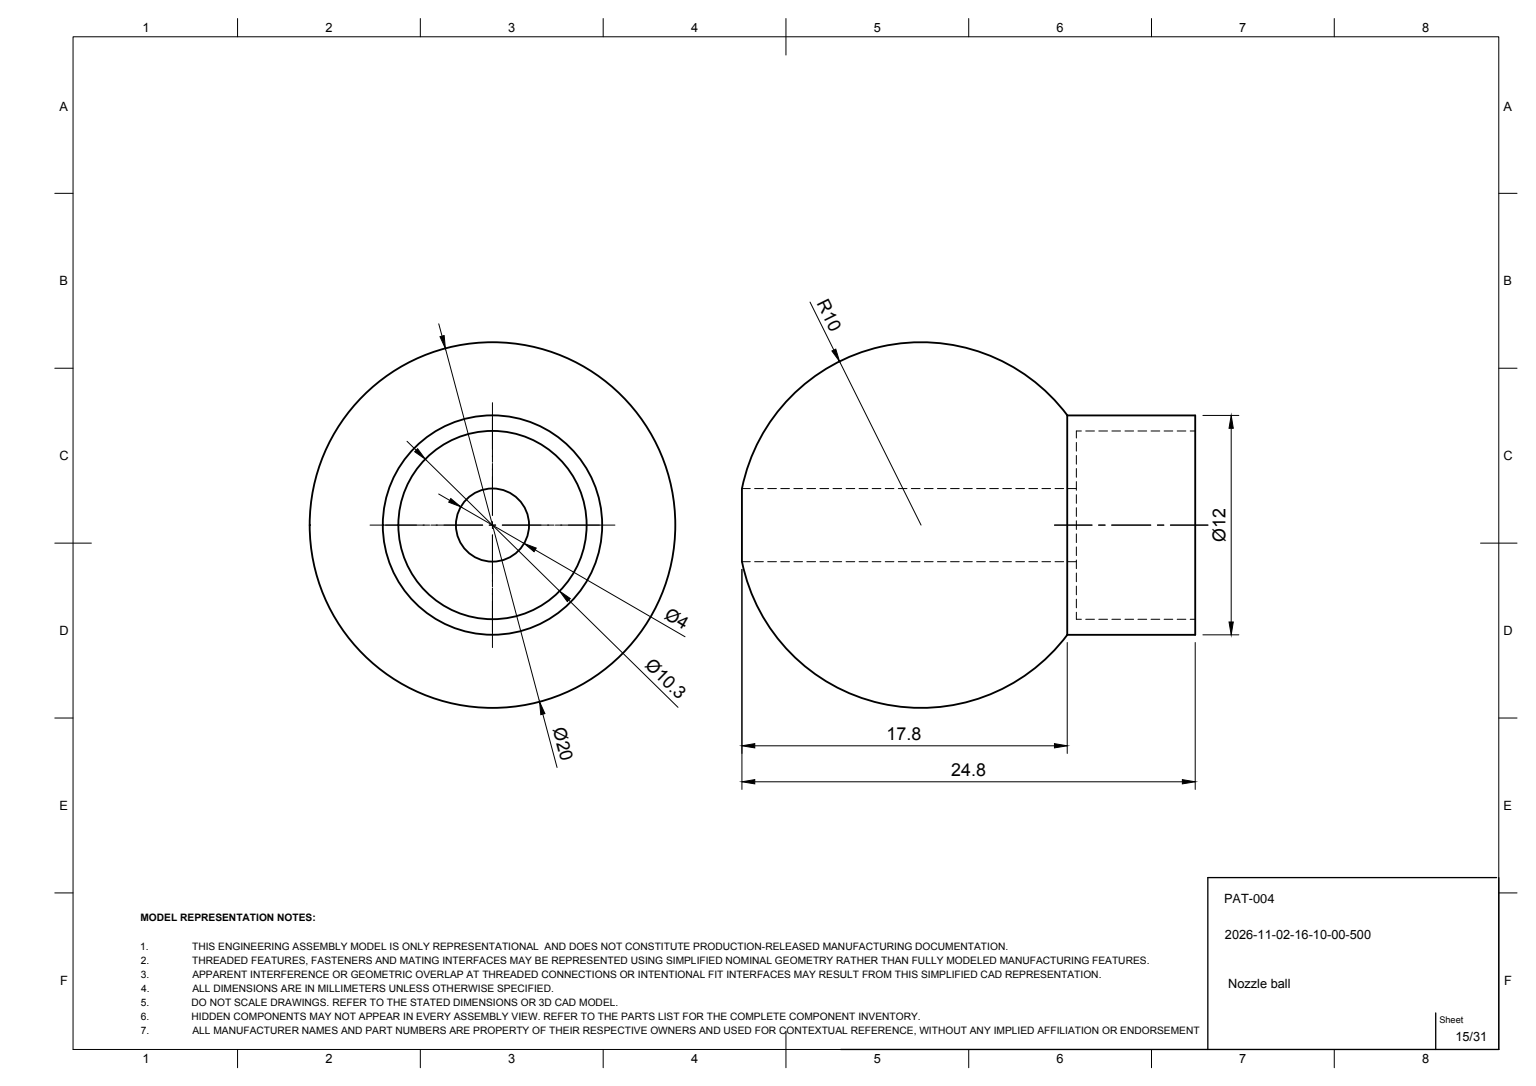
ISO-10303-21;
HEADER;
/* Generated by software containing ST-Developer
 * from STEP Tools, Inc. (www.steptools.com) 
 */

FILE_DESCRIPTION(
/* description */ ('Air blow-off nozzle station'),
/* implementation_level */ '2;1');

FILE_NAME(
/* name */ 'Nozzle ball.step',
/* time_stamp */ '2026-10-27T10:53:54-07:00',
/* author */ (''),
/* organization */ (''),
/* preprocessor_version */ 'ST-DEVELOPER v20.2',
/* originating_system */ 'Autodesk Translation Framework v15.17.0.0',
/* authorisation */ '');

FILE_SCHEMA (('AUTOMOTIVE_DESIGN { 1 0 10303 214 3 1 1 }'));
ENDSEC;

DATA;
#10=MECHANICAL_DESIGN_GEOMETRIC_PRESENTATION_REPRESENTATION('',(#251),#7897);
#168=SPHERICAL_SURFACE('',#4914,1.);
#201=SHAPE_REPRESENTATION_RELATIONSHIP('SRR','None',#8016,#226);
#226=ADVANCED_BREP_SHAPE_REPRESENTATION('',(#274),#7883);
#251=STYLED_ITEM('',(#8234),#274);
#274=MANIFOLD_SOLID_BREP('Body1',#4302);
#335=FACE_BOUND('',#1033,.T.);
#336=FACE_BOUND('',#1037,.T.);
#337=FACE_BOUND('',#1039,.T.);
#338=FACE_BOUND('',#1040,.T.);
#504=PLANE('',#4906);
#505=PLANE('',#4913);
#725=FACE_OUTER_BOUND('',#1031,.T.);
#726=FACE_OUTER_BOUND('',#1032,.T.);
#727=FACE_OUTER_BOUND('',#1034,.T.);
#728=FACE_OUTER_BOUND('',#1035,.T.);
#729=FACE_OUTER_BOUND('',#1036,.T.);
#730=FACE_OUTER_BOUND('',#1038,.T.);
#1031=EDGE_LOOP('',(#3725,#3726,#3727,#3728));
#1032=EDGE_LOOP('',(#3729));
#1033=EDGE_LOOP('',(#3730));
#1034=EDGE_LOOP('',(#3731,#3732,#3733,#3734));
#1035=EDGE_LOOP('',(#3735,#3736,#3737,#3738));
#1036=EDGE_LOOP('',(#3739));
#1037=EDGE_LOOP('',(#3740));
#1038=EDGE_LOOP('',(#3741,#3742));
#1039=EDGE_LOOP('',(#3743));
#1040=EDGE_LOOP('',(#3744));
#1442=LINE('',#7537,#1796);
#1443=LINE('',#7544,#1797);
#1444=LINE('',#7550,#1798);
#1796=VECTOR('',#6008,0.515);
#1797=VECTOR('',#6017,0.2);
#1798=VECTOR('',#6024,0.6);
#1940=CIRCLE('',#4904,0.515);
#1941=CIRCLE('',#4905,0.515);
#1942=CIRCLE('',#4907,0.2);
#1943=CIRCLE('',#4909,0.2);
#1944=CIRCLE('',#4911,0.6);
#1945=CIRCLE('',#4912,0.6);
#1946=CIRCLE('',#4915,1.);
#2284=VERTEX_POINT('',#7534);
#2285=VERTEX_POINT('',#7536);
#2286=VERTEX_POINT('',#7540);
#2287=VERTEX_POINT('',#7543);
#2288=VERTEX_POINT('',#7547);
#2289=VERTEX_POINT('',#7549);
#2290=VERTEX_POINT('',#7554);
#2291=VERTEX_POINT('',#7555);
#2780=EDGE_CURVE('',#2284,#2284,#1940,.T.);
#2781=EDGE_CURVE('',#2284,#2285,#1442,.T.);
#2782=EDGE_CURVE('',#2285,#2285,#1941,.T.);
#2783=EDGE_CURVE('',#2286,#2286,#1942,.T.);
#2784=EDGE_CURVE('',#2286,#2287,#1443,.T.);
#2785=EDGE_CURVE('',#2287,#2287,#1943,.T.);
#2786=EDGE_CURVE('',#2288,#2288,#1944,.T.);
#2787=EDGE_CURVE('',#2288,#2289,#1444,.T.);
#2788=EDGE_CURVE('',#2289,#2289,#1945,.T.);
#2789=EDGE_CURVE('',#2290,#2291,#1946,.T.);
#3725=ORIENTED_EDGE('',*,*,#2780,.F.);
#3726=ORIENTED_EDGE('',*,*,#2781,.T.);
#3727=ORIENTED_EDGE('',*,*,#2782,.T.);
#3728=ORIENTED_EDGE('',*,*,#2781,.F.);
#3729=ORIENTED_EDGE('',*,*,#2782,.F.);
#3730=ORIENTED_EDGE('',*,*,#2783,.F.);
#3731=ORIENTED_EDGE('',*,*,#2783,.T.);
#3732=ORIENTED_EDGE('',*,*,#2784,.T.);
#3733=ORIENTED_EDGE('',*,*,#2785,.F.);
#3734=ORIENTED_EDGE('',*,*,#2784,.F.);
#3735=ORIENTED_EDGE('',*,*,#2786,.F.);
#3736=ORIENTED_EDGE('',*,*,#2787,.T.);
#3737=ORIENTED_EDGE('',*,*,#2788,.T.);
#3738=ORIENTED_EDGE('',*,*,#2787,.F.);
#3739=ORIENTED_EDGE('',*,*,#2788,.F.);
#3740=ORIENTED_EDGE('',*,*,#2780,.T.);
#3741=ORIENTED_EDGE('',*,*,#2789,.T.);
#3742=ORIENTED_EDGE('',*,*,#2789,.F.);
#3743=ORIENTED_EDGE('',*,*,#2785,.T.);
#3744=ORIENTED_EDGE('',*,*,#2786,.T.);
#3998=CYLINDRICAL_SURFACE('',#4903,0.515);
#3999=CYLINDRICAL_SURFACE('',#4908,0.2);
#4000=CYLINDRICAL_SURFACE('',#4910,0.6);
#4215=ADVANCED_FACE('',(#725),#3998,.F.);
#4216=ADVANCED_FACE('',(#726,#335),#504,.F.);
#4217=ADVANCED_FACE('',(#727),#3999,.F.);
#4218=ADVANCED_FACE('',(#728),#4000,.T.);
#4219=ADVANCED_FACE('',(#729,#336),#505,.F.);
#4220=ADVANCED_FACE('',(#730,#337,#338),#168,.T.);
#4302=CLOSED_SHELL('',(#4215,#4216,#4217,#4218,#4219,#4220));
#4902=AXIS2_PLACEMENT_3D('',#7532,#6002,#6003);
#4903=AXIS2_PLACEMENT_3D('',#7533,#6004,#6005);
#4904=AXIS2_PLACEMENT_3D('',#7535,#6006,#6007);
#4905=AXIS2_PLACEMENT_3D('',#7538,#6009,#6010);
#4906=AXIS2_PLACEMENT_3D('',#7539,#6011,#6012);
#4907=AXIS2_PLACEMENT_3D('',#7541,#6013,#6014);
#4908=AXIS2_PLACEMENT_3D('',#7542,#6015,#6016);
#4909=AXIS2_PLACEMENT_3D('',#7545,#6018,#6019);
#4910=AXIS2_PLACEMENT_3D('',#7546,#6020,#6021);
#4911=AXIS2_PLACEMENT_3D('',#7548,#6022,#6023);
#4912=AXIS2_PLACEMENT_3D('',#7551,#6025,#6026);
#4913=AXIS2_PLACEMENT_3D('',#7552,#6027,#6028);
#4914=AXIS2_PLACEMENT_3D('',#7553,#6029,#6030);
#4915=AXIS2_PLACEMENT_3D('',#7556,#6031,#6032);
#6002=DIRECTION('axis',(0.,0.,1.));
#6003=DIRECTION('refdir',(1.,0.,0.));
#6004=DIRECTION('center_axis',(0.,1.,0.));
#6005=DIRECTION('ref_axis',(1.,0.,0.));
#6006=DIRECTION('center_axis',(0.,1.,0.));
#6007=DIRECTION('ref_axis',(1.,0.,0.));
#6008=DIRECTION('',(0.,1.,0.));
#6009=DIRECTION('center_axis',(0.,1.,0.));
#6010=DIRECTION('ref_axis',(1.,0.,0.));
#6011=DIRECTION('center_axis',(0.,1.,0.));
#6012=DIRECTION('ref_axis',(1.,0.,0.));
#6013=DIRECTION('center_axis',(0.,-1.,0.));
#6014=DIRECTION('ref_axis',(1.,0.,0.));
#6015=DIRECTION('center_axis',(0.,1.,0.));
#6016=DIRECTION('ref_axis',(1.,0.,0.));
#6017=DIRECTION('',(0.,1.,0.));
#6018=DIRECTION('center_axis',(0.,-1.,0.));
#6019=DIRECTION('ref_axis',(1.,-1.11022302462516E-15,0.));
#6020=DIRECTION('center_axis',(0.,1.,0.));
#6021=DIRECTION('ref_axis',(1.,0.,0.));
#6022=DIRECTION('center_axis',(0.,1.,0.));
#6023=DIRECTION('ref_axis',(1.,0.,0.));
#6024=DIRECTION('',(0.,-1.,0.));
#6025=DIRECTION('center_axis',(0.,1.,0.));
#6026=DIRECTION('ref_axis',(1.,0.,0.));
#6027=DIRECTION('center_axis',(0.,1.,0.));
#6028=DIRECTION('ref_axis',(1.,0.,0.));
#6029=DIRECTION('center_axis',(0.,0.,1.));
#6030=DIRECTION('ref_axis',(1.,0.,0.));
#6031=DIRECTION('center_axis',(0.,-1.,0.));
#6032=DIRECTION('ref_axis',(-1.,0.,0.));
#7532=CARTESIAN_POINT('',(0.,0.,0.));
#7533=CARTESIAN_POINT('Origin',(-3.,-3.6,23.));
#7534=CARTESIAN_POINT('',(-3.515,-3.5,23.));
#7535=CARTESIAN_POINT('Origin',(-3.,-3.5,23.));
#7536=CARTESIAN_POINT('',(-3.515,-2.85,23.));
#7537=CARTESIAN_POINT('',(-3.515,-3.6,23.));
#7538=CARTESIAN_POINT('Origin',(-3.,-2.85,23.));
#7539=CARTESIAN_POINT('Origin',(-3.,-2.85,23.));
#7540=CARTESIAN_POINT('',(-3.2,-2.85,23.));
#7541=CARTESIAN_POINT('Origin',(-3.,-2.85,23.));
#7542=CARTESIAN_POINT('Origin',(-3.,-3.6,23.));
#7543=CARTESIAN_POINT('',(-3.2,-1.02020410288673,23.));
#7544=CARTESIAN_POINT('',(-3.2,-3.6,23.));
#7545=CARTESIAN_POINT('Origin',(-3.,-1.02020410288673,23.));
#7546=CARTESIAN_POINT('Origin',(-3.,-3.5,23.));
#7547=CARTESIAN_POINT('',(-3.6,-2.8,23.));
#7548=CARTESIAN_POINT('Origin',(-3.,-2.8,23.));
#7549=CARTESIAN_POINT('',(-3.6,-3.5,23.));
#7550=CARTESIAN_POINT('',(-3.6,-3.5,23.));
#7551=CARTESIAN_POINT('Origin',(-3.,-3.5,23.));
#7552=CARTESIAN_POINT('Origin',(-3.,-3.5,23.));
#7553=CARTESIAN_POINT('Origin',(-3.,-2.,23.));
#7554=CARTESIAN_POINT('',(-3.,-2.,24.));
#7555=CARTESIAN_POINT('',(-3.,-2.,22.));
#7556=CARTESIAN_POINT('Origin',(-3.,-2.,23.));
#7851=UNCERTAINTY_MEASURE_WITH_UNIT(LENGTH_MEASURE(0.001),#7898,
'DISTANCE_ACCURACY_VALUE',
'Maximum model space distance between geometric entities at asserted c
onnectivities');
#7865=UNCERTAINTY_MEASURE_WITH_UNIT(LENGTH_MEASURE(0.001),#7898,
'DISTANCE_ACCURACY_VALUE',
'Maximum model space distance between geometric entities at asserted c
onnectivities');
#7883=(
GEOMETRIC_REPRESENTATION_CONTEXT(3)
GLOBAL_UNCERTAINTY_ASSIGNED_CONTEXT((#7851))
GLOBAL_UNIT_ASSIGNED_CONTEXT((#7898,#7900,#7901))
REPRESENTATION_CONTEXT('','3D')
);
#7897=(
GEOMETRIC_REPRESENTATION_CONTEXT(3)
GLOBAL_UNCERTAINTY_ASSIGNED_CONTEXT((#7865))
GLOBAL_UNIT_ASSIGNED_CONTEXT((#7898,#7900,#7901))
REPRESENTATION_CONTEXT('','3D')
);
#7898=(
LENGTH_UNIT()
NAMED_UNIT(*)
SI_UNIT(.CENTI.,.METRE.)
);
#7900=(
NAMED_UNIT(*)
PLANE_ANGLE_UNIT()
SI_UNIT($,.RADIAN.)
);
#7901=(
NAMED_UNIT(*)
SI_UNIT($,.STERADIAN.)
SOLID_ANGLE_UNIT()
);
#7919=SHAPE_DEFINITION_REPRESENTATION(#7967,#8016);
#7967=PRODUCT_DEFINITION_SHAPE('',$,#8048);
#8016=SHAPE_REPRESENTATION('',(#4902),#7883);
#8030=PRODUCT_DEFINITION_CONTEXT('part definition',#8125,'design');
#8048=PRODUCT_DEFINITION('Nozzle ball','Nozzle ball',#8079,#8030);
#8079=PRODUCT_DEFINITION_FORMATION('',$,#8144);
#8125=APPLICATION_CONTEXT(
'Core Data for Automotive Mechanical Design Process');
#8126=PRODUCT_CONTEXT('part definition',#8125,'mechanical');
#8144=PRODUCT('Nozzle ball','Nozzle ball','Nozzle ball',(#8126));
#8228=COLOUR_RGB('Off White',0.89,0.88,0.83);
#8229=FILL_AREA_STYLE_COLOUR('',#8228);
#8230=FILL_AREA_STYLE('',(#8229));
#8231=SURFACE_STYLE_FILL_AREA(#8230);
#8232=SURFACE_SIDE_STYLE('',(#8231));
#8233=SURFACE_STYLE_USAGE(.BOTH.,#8232);
#8234=PRESENTATION_STYLE_ASSIGNMENT((#8233));
ENDSEC;
END-ISO-10303-21;
